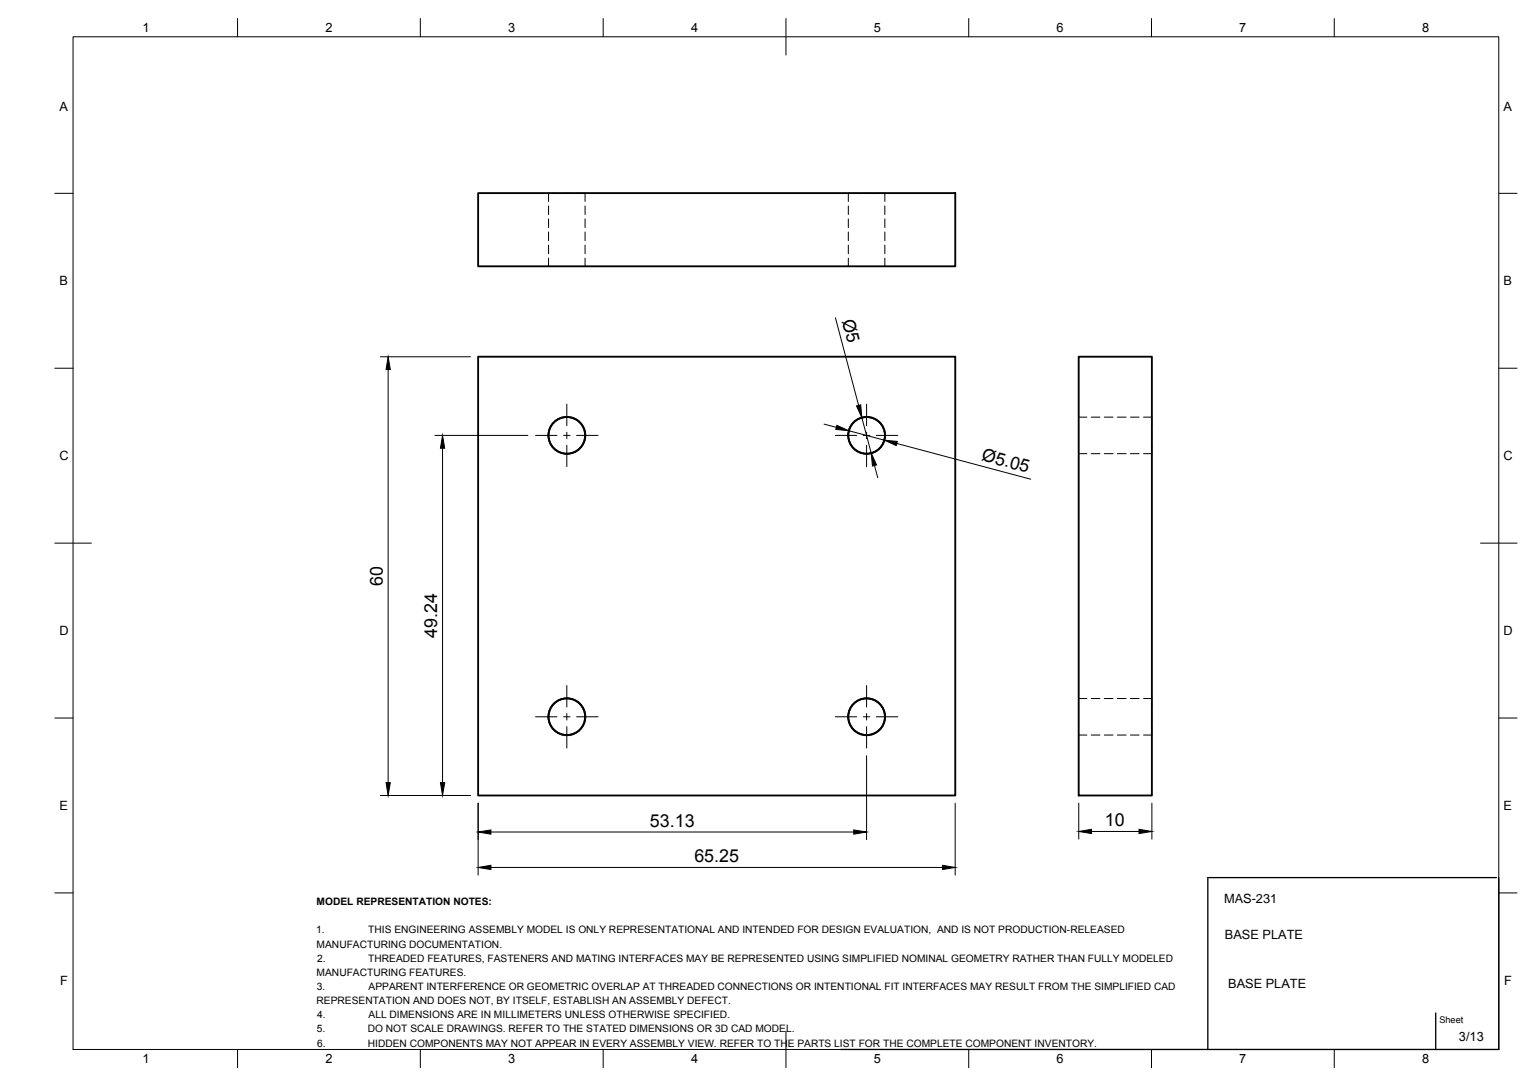
ISO-10303-21;
HEADER;
FILE_DESCRIPTION (('STEP AP214'),
    '1' );
FILE_NAME ( 'Base Plate.step', '2026-10-04T02:08:54', ( '' ), ( '' ), 'STEP AP214', 'Unspecified', '' );
FILE_SCHEMA (( 'AUTOMOTIVE_DESIGN' ));
ENDSEC;
DATA;
#315=EDGE_CURVE ( 'NONE', #5716, #5360, #10980, .T. ) ;
#330=AXIS2_PLACEMENT_3D ( 'NONE', #15898, #1005, #37686 ) ;
#400=CONICAL_SURFACE ( 'NONE', #29553, 0.09842519685039310962, 0.7853981633972314524 ) ;
#581=AXIS2_PLACEMENT_3D ( 'NONE', #37868, #23494, #19160 ) ;
#651=ORIENTED_EDGE ( 'NONE', *, *, #28716, .F. ) ;
#675=DIRECTION ( 'NONE',  ( 0.000000000000000000, 1.000000000000000000, 0.000000000000000000 ) ) ;
#805=AXIS2_PLACEMENT_3D ( 'NONE', #34915, #9017, #31319 ) ;
#889=CARTESIAN_POINT ( 'NONE',  ( 0.8070866141732283561, -0.0009842519685049383633, 0.8559055118110230342 ) ) ;
#932=ORIENTED_EDGE ( 'NONE', *, *, #10243, .T. ) ;
#978=PLANE ( 'NONE',  #26301 ) ;
#991=DIRECTION ( 'NONE',  ( 0.000000000000000000, 1.000000000000000000, 0.000000000000000000 ) ) ;
#1005=DIRECTION ( 'NONE',  ( 0.000000000000000000, 1.000000000000000000, 0.000000000000000000 ) ) ;
#1050=ORIENTED_EDGE ( 'NONE', *, *, #18714, .T. ) ;
#1080=CONICAL_SURFACE ( 'NONE', #330, 0.09842519685039310962, 0.7853981633972314524 ) ;
#1170=VERTEX_POINT ( 'NONE', #7542 ) ;
#1242=VERTEX_POINT ( 'NONE', #23759 ) ;
#1252=EDGE_LOOP ( 'NONE', ( #11130, #15694, #34141, #24810 ) ) ;
#1459=FACE_OUTER_BOUND ( 'NONE', #19089, .T. ) ;
#1546=EDGE_LOOP ( 'NONE', ( #9201, #4846, #43494, #46692 ) ) ;
#1588=ORIENTED_EDGE ( 'NONE', *, *, #46677, .T. ) ;
#1771=DIRECTION ( 'NONE',  ( 0.000000000000000000, 0.000000000000000000, 1.000000000000000000 ) ) ;
#1848=ADVANCED_FACE ( 'NONE', ( #21708 ), #3242, .F. ) ;
#1945=CONICAL_SURFACE ( 'NONE', #26464, 0.09842519685039310962, 0.7853981633972314524 ) ;
#2206=FACE_OUTER_BOUND ( 'NONE', #4838, .T. ) ;
#2223=CARTESIAN_POINT ( 'NONE',  ( 0.8070866141732283561, 0.000000000000000000, 0.7574803149606299524 ) ) ;
#2287=ORIENTED_EDGE ( 'NONE', *, *, #20440, .F. ) ;
#2478=PRODUCT_DEFINITION_CONTEXT ( 'detailed design', #11336, 'design' ) ;
#2480=VERTEX_POINT ( 'NONE', #27806 ) ;
#2571=LINE ( 'NONE', #39233, #13199 ) ;
#2637=ORIENTED_EDGE ( 'NONE', *, *, #8911, .F. ) ;
#2705=ORIENTED_EDGE ( 'NONE', *, *, #4811, .F. ) ;
#2813=DIRECTION ( 'NONE',  ( 0.000000000000000000, 1.000000000000000000, 0.000000000000000000 ) ) ;
#3034=ORIENTED_EDGE ( 'NONE', *, *, #40501, .T. ) ;
#3242=CYLINDRICAL_SURFACE ( 'NONE', #18362, 0.09842519685039310962 ) ;
#3388=( NAMED_UNIT ( * ) SI_UNIT ( $, .STERADIAN. ) SOLID_ANGLE_UNIT ( ) ) ;
#3451=ORIENTED_EDGE ( 'NONE', *, *, #11714, .F. ) ;
#3490=EDGE_LOOP ( 'NONE', ( #8008, #46438, #11694, #3034 ) ) ;
#3519=EDGE_CURVE ( 'NONE', #10456, #24872, #30387, .T. ) ;
#3675=CIRCLE ( 'NONE', #41893, 0.09842519685039310962 ) ;
#3812=FACE_BOUND ( 'NONE', #17412, .T. ) ;
#3834=VERTEX_POINT ( 'NONE', #35885 ) ;
#3929=DIRECTION ( 'NONE',  ( 0.000000000000000000, 1.000000000000000000, 0.000000000000000000 ) ) ;
#3941=LENGTH_MEASURE_WITH_UNIT ( LENGTH_MEASURE( 0.02539999999999999897 ), #37017 ) ;
#3945=DIRECTION ( 'NONE',  ( 0.000000000000000000, 0.000000000000000000, 1.000000000000000000 ) ) ;
#4069=DIRECTION ( 'NONE',  ( 0.000000000000000000, 0.000000000000000000, 1.000000000000000000 ) ) ;
#4078=DIRECTION ( 'NONE',  ( 0.000000000000000000, 0.7071067811867007835, 0.7071067811863941399 ) ) ;
#4150=EDGE_CURVE ( 'NONE', #1170, #31291, #25492, .T. ) ;
#4170=EDGE_LOOP ( 'NONE', ( #24125, #6496, #36526, #10576 ) ) ;
#4195=CIRCLE ( 'NONE', #42468, 0.09940944881889761386 ) ;
#4286=CARTESIAN_POINT ( 'NONE',  ( -1.284448818897637956, -0.3937007874015748254, -1.181102362204724310 ) ) ;
#4382=CARTESIAN_POINT ( 'NONE',  ( 0.8070866141732283561, -0.0009842519685049383633, -0.7574803149606299524 ) ) ;
#4481=AXIS2_PLACEMENT_3D ( 'NONE', #6050, #17084, #13724 ) ;
#4668=EDGE_LOOP ( 'NONE', ( #34347, #651, #38280, #27775 ) ) ;
#4787=CARTESIAN_POINT ( 'NONE',  ( 0.8070866141732283561, -0.0009842519685049383633, -0.8559055118110230342 ) ) ;
#4811=EDGE_CURVE ( 'NONE', #11722, #39584, #46217, .T. ) ;
#4815=DIRECTION ( 'NONE',  ( 1.000000000000000000, -0.000000000000000000, 0.000000000000000000 ) ) ;
#4832=ORIENTED_EDGE ( 'NONE', *, *, #8571, .T. ) ;
#4838=EDGE_LOOP ( 'NONE', ( #34045, #33951, #29727, #22816 ) ) ;
#4846=ORIENTED_EDGE ( 'NONE', *, *, #40501, .F. ) ;
#5141=AXIS2_PLACEMENT_3D ( 'NONE', #9800, #39013, #35676 ) ;
#5145=DIRECTION ( 'NONE',  ( 0.000000000000000000, 1.000000000000000000, 0.000000000000000000 ) ) ;
#5205=ORIENTED_EDGE ( 'NONE', *, *, #25069, .F. ) ;
#5271=CIRCLE ( 'NONE', #26704, 0.09842519685039310962 ) ;
#5360=VERTEX_POINT ( 'NONE', #7812 ) ;
#5579=DIRECTION ( 'NONE',  ( -1.000000000000000000, 0.000000000000000000, 0.000000000000000000 ) ) ;
#5587=AXIS2_PLACEMENT_3D ( 'NONE', #43394, #39329, #25205 ) ;
#5634=DIRECTION ( 'NONE',  ( 0.000000000000000000, 1.000000000000000000, 0.000000000000000000 ) ) ;
#5716=VERTEX_POINT ( 'NONE', #40952 ) ;
#5744=EDGE_CURVE ( 'NONE', #31115, #24872, #37874, .T. ) ;
#5913=EDGE_CURVE ( 'NONE', #14452, #1242, #11460, .T. ) ;
#5977=ADVANCED_FACE ( 'NONE', ( #11706, #44963, #26331, #40892, #22950 ), #18632, .T. ) ;
#6029=DIRECTION ( 'NONE',  ( 0.000000000000000000, 0.000000000000000000, 1.000000000000000000 ) ) ;
#6050=CARTESIAN_POINT ( 'NONE',  ( 0.8070866141732283561, -0.0009842519685049383633, 0.7574803149606299524 ) ) ;
#6143=AXIS2_PLACEMENT_3D ( 'NONE', #30741, #991, #12283 ) ;
#6148=CIRCLE ( 'NONE', #39801, 0.09842519685039310962 ) ;
#6493=ADVANCED_FACE ( 'NONE', ( #34883 ), #1945, .F. ) ;
#6496=ORIENTED_EDGE ( 'NONE', *, *, #25069, .T. ) ;
#6566=VECTOR ( 'NONE', #5579, 39.37007874015748143 ) ;
#6588=DIRECTION ( 'NONE',  ( 0.000000000000000000, 0.000000000000000000, 1.000000000000000000 ) ) ;
#6628=LINE ( 'NONE', #21244, #26508 ) ;
#6675=AXIS2_PLACEMENT_3D ( 'NONE', #36792, #26011, #3945 ) ;
#6892=DIRECTION ( 'NONE',  ( -0.000000000000000000, 1.000000000000000000, -0.000000000000000000 ) ) ;
#7281=DIRECTION ( 'NONE',  ( 0.000000000000000000, 0.000000000000000000, 1.000000000000000000 ) ) ;
#7289=AXIS2_PLACEMENT_3D ( 'NONE', #7614, #32821, #25133 ) ;
#7317=PRODUCT_DEFINITION_SHAPE ( 'NONE', 'NONE',  #36823 ) ;
#7358=FACE_OUTER_BOUND ( 'NONE', #30567, .T. ) ;
#7396=CARTESIAN_POINT ( 'NONE',  ( 0.8070866141732283561, 0.000000000000000000, -0.7574803149606299524 ) ) ;
#7494=ORIENTED_EDGE ( 'NONE', *, *, #46842, .T. ) ;
#7530=CIRCLE ( 'NONE', #20536, 0.09842519685039310962 ) ;
#7542=CARTESIAN_POINT ( 'NONE',  ( -0.8070866141732283561, -0.3937007874015746034, -0.8559055118110230342 ) ) ;
#7568=ADVANCED_FACE ( 'NONE', ( #11132 ), #22840, .T. ) ;
#7614=CARTESIAN_POINT ( 'NONE',  ( -0.8070866141732283561, 0.000000000000000000, 0.7574803149606299524 ) ) ;
#7634=FACE_OUTER_BOUND ( 'NONE', #45486, .T. ) ;
#7663=AXIS2_PLACEMENT_3D ( 'NONE', #26053, #29917, #8526 ) ;
#7737=FACE_OUTER_BOUND ( 'NONE', #25691, .T. ) ;
#7797=EDGE_CURVE ( 'NONE', #28803, #31115, #8610, .T. ) ;
#7798=LINE ( 'NONE', #18816, #17656 ) ;
#7812=CARTESIAN_POINT ( 'NONE',  ( -0.8070866141732283561, 0.000000000000000000, 0.6580708661417323802 ) ) ;
#7880=DIRECTION ( 'NONE',  ( -0.000000000000000000, 1.000000000000000000, 0.000000000000000000 ) ) ;
#7901=EDGE_CURVE ( 'NONE', #15275, #1242, #11102, .T. ) ;
#7933=CARTESIAN_POINT ( 'NONE',  ( 0.8070866141732283561, -0.0009842519685049383633, 0.8559055118110230342 ) ) ;
#8000=CARTESIAN_POINT ( 'NONE',  ( -0.8070866141732283561, 0.000000000000000000, -0.7574803149606299524 ) ) ;
#8008=ORIENTED_EDGE ( 'NONE', *, *, #26812, .F. ) ;
#8058=CARTESIAN_POINT ( 'NONE',  ( 1.284448818897637956, 0.000000000000000000, -1.181102362204724310 ) ) ;
#8059=EDGE_CURVE ( 'NONE', #39837, #14452, #41653, .T. ) ;
#8115=PLANE ( 'NONE',  #11348 ) ;
#8130=UNCERTAINTY_MEASURE_WITH_UNIT (LENGTH_MEASURE( 1.000000000000000082E-05 ), #44890, 'distance_accuracy_value', 'NONE') ;
#8136=DIRECTION ( 'NONE',  ( 0.000000000000000000, 0.000000000000000000, 1.000000000000000000 ) ) ;
#8448=AXIS2_PLACEMENT_3D ( 'NONE', #2223, #41983, #20909 ) ;
#8526=DIRECTION ( 'NONE',  ( 0.000000000000000000, 0.000000000000000000, 1.000000000000000000 ) ) ;
#8571=EDGE_CURVE ( 'NONE', #26504, #25961, #12011, .T. ) ;
#8610=LINE ( 'NONE', #4286, #20278 ) ;
#8677=FACE_OUTER_BOUND ( 'NONE', #35087, .T. ) ;
#8853=ORIENTED_EDGE ( 'NONE', *, *, #11923, .F. ) ;
#8911=EDGE_CURVE ( 'NONE', #25961, #37257, #29546, .T. ) ;
#9017=DIRECTION ( 'NONE',  ( -0.000000000000000000, 1.000000000000000000, -0.000000000000000000 ) ) ;
#9047=ADVANCED_FACE ( 'NONE', ( #25850 ), #40433, .F. ) ;
#9136=DIRECTION ( 'NONE',  ( -0.000000000000000000, 1.000000000000000000, -0.000000000000000000 ) ) ;
#9137=AXIS2_PLACEMENT_3D ( 'NONE', #36669, #14627, #21570 ) ;
#9201=ORIENTED_EDGE ( 'NONE', *, *, #27851, .F. ) ;
#9223=AXIS2_PLACEMENT_3D ( 'NONE', #8000, #18549, #29403 ) ;
#9407=ORIENTED_EDGE ( 'NONE', *, *, #4150, .F. ) ;
#9658=SHAPE_DEFINITION_REPRESENTATION ( #7317, #30762 ) ;
#9710=EDGE_CURVE ( 'NONE', #18061, #11722, #40144, .T. ) ;
#9759=DIRECTION ( 'NONE',  ( 0.000000000000000000, 0.000000000000000000, -1.000000000000000000 ) ) ;
#9800=CARTESIAN_POINT ( 'NONE',  ( 0.8070866141732283561, -0.0009842519685049383633, 0.7574803149606299524 ) ) ;
#9852=ORIENTED_EDGE ( 'NONE', *, *, #7901, .F. ) ;
#10204=CARTESIAN_POINT ( 'NONE',  ( 0.8070866141732283561, -0.3937007874015746034, -0.7574803149606299524 ) ) ;
#10243=EDGE_CURVE ( 'NONE', #44955, #14452, #31944, .T. ) ;
#10358=EDGE_LOOP ( 'NONE', ( #22529, #42334, #12122, #27521 ) ) ;
#10359=EDGE_CURVE ( 'NONE', #22756, #27408, #46200, .T. ) ;
#10456=VERTEX_POINT ( 'NONE', #22399 ) ;
#10576=ORIENTED_EDGE ( 'NONE', *, *, #46842, .F. ) ;
#10585=CARTESIAN_POINT ( 'NONE',  ( -0.8070866141732283561, -0.3937007874015746034, 0.7574803149606299524 ) ) ;
#10681=EDGE_CURVE ( 'NONE', #20094, #24250, #43403, .T. ) ;
#10719=DIRECTION ( 'NONE',  ( 8.659560562353054383E-17, 0.7071067811867007835, -0.7071067811863941399 ) ) ;
#10725=EDGE_CURVE ( 'NONE', #22756, #28803, #40345, .T. ) ;
#10805=MECHANICAL_DESIGN_GEOMETRIC_PRESENTATION_REPRESENTATION('',(#19186),#41362);
#10835=DIRECTION ( 'NONE',  ( 1.000000000000000000, 0.000000000000000000, 0.000000000000000000 ) ) ;
#10869=DIRECTION ( 'NONE',  ( 0.000000000000000000, 0.000000000000000000, 1.000000000000000000 ) ) ;
#10980=CIRCLE ( 'NONE', #37859, 0.09940944881889761386 ) ;
#11020=DIRECTION ( 'NONE',  ( 8.659560562353054383E-17, 0.7071067811867007835, -0.7071067811863941399 ) ) ;
#11049=ORIENTED_EDGE ( 'NONE', *, *, #43540, .F. ) ;
#11074=EDGE_CURVE ( 'NONE', #29015, #39837, #11313, .T. ) ;
#11102=CIRCLE ( 'NONE', #43217, 0.09940944881889761386 ) ;
#11130=ORIENTED_EDGE ( 'NONE', *, *, #20351, .F. ) ;
#11132=FACE_OUTER_BOUND ( 'NONE', #12538, .T. ) ;
#11176=ORIENTED_EDGE ( 'NONE', *, *, #19700, .F. ) ;
#11220=CARTESIAN_POINT ( 'NONE',  ( 0.8070866141732283561, 0.000000000000000000, 0.8559055118110230342 ) ) ;
#11313=CIRCLE ( 'NONE', #6675, 0.09842519685039310962 ) ;
#11336=APPLICATION_CONTEXT ( 'automotive_design' ) ;
#11348=AXIS2_PLACEMENT_3D ( 'NONE', #33797, #7880, #15576 ) ;
#11385=CARTESIAN_POINT ( 'NONE',  ( 1.284448818897637956, -0.3937007874015748254, -1.181102362204724310 ) ) ;
#11450=AXIS2_PLACEMENT_3D ( 'NONE', #22352, #13997, #7281 ) ;
#11460=LINE ( 'NONE', #25845, #21062 ) ;
#11694=ORIENTED_EDGE ( 'NONE', *, *, #16527, .T. ) ;
#11706=FACE_BOUND ( 'NONE', #31447, .T. ) ;
#11714=EDGE_CURVE ( 'NONE', #32806, #13348, #3675, .T. ) ;
#11722=VERTEX_POINT ( 'NONE', #43133 ) ;
#11838=LINE ( 'NONE', #34587, #6566 ) ;
#11889=VECTOR ( 'NONE', #14058, 39.37007874015748143 ) ;
#11923=EDGE_CURVE ( 'NONE', #26504, #47218, #15149, .T. ) ;
#11943=FACE_OUTER_BOUND ( 'NONE', #3490, .T. ) ;
#12011=LINE ( 'NONE', #4787, #14204 ) ;
#12089=ORIENTED_EDGE ( 'NONE', *, *, #8059, .F. ) ;
#12122=ORIENTED_EDGE ( 'NONE', *, *, #17641, .T. ) ;
#12174=DIRECTION ( 'NONE',  ( -0.000000000000000000, 1.000000000000000000, 0.000000000000000000 ) ) ;
#12192=CARTESIAN_POINT ( 'NONE',  ( -0.8070866141732283561, -0.0009842519685049383633, 0.8559055118110230342 ) ) ;
#12197=CYLINDRICAL_SURFACE ( 'NONE', #24627, 0.09842519685039310962 ) ;
#12201=EDGE_CURVE ( 'NONE', #36286, #31518, #7530, .T. ) ;
#12283=DIRECTION ( 'NONE',  ( 0.000000000000000000, 0.000000000000000000, 1.000000000000000000 ) ) ;
#12373=ORIENTED_EDGE ( 'NONE', *, *, #22828, .F. ) ;
#12375=EDGE_CURVE ( 'NONE', #47218, #37257, #18468, .T. ) ;
#12379=AXIS2_PLACEMENT_3D ( 'NONE', #32536, #33483, #25809 ) ;
#12420=AXIS2_PLACEMENT_3D ( 'NONE', #32416, #39325, #14656 ) ;
#12507=DIRECTION ( 'NONE',  ( 0.000000000000000000, 0.7071067811867007835, 0.7071067811863941399 ) ) ;
#12538=EDGE_LOOP ( 'NONE', ( #42275, #17973, #13010, #43115 ) ) ;
#12632=DIRECTION ( 'NONE',  ( 0.000000000000000000, 0.000000000000000000, -1.000000000000000000 ) ) ;
#12979=CARTESIAN_POINT ( 'NONE',  ( 1.284448818897637956, -0.3937007874015748254, 1.181102362204724310 ) ) ;
#13010=ORIENTED_EDGE ( 'NONE', *, *, #10725, .T. ) ;
#13076=ORIENTED_EDGE ( 'NONE', *, *, #8911, .T. ) ;
#13199=VECTOR ( 'NONE', #38781, 39.37007874015748143 ) ;
#13203=CIRCLE ( 'NONE', #45310, 0.09940944881889761386 ) ;
#13257=CYLINDRICAL_SURFACE ( 'NONE', #24915, 0.09842519685039310962 ) ;
#13309=EDGE_LOOP ( 'NONE', ( #34696, #24463, #14277, #2705 ) ) ;
#13348=VERTEX_POINT ( 'NONE', #24149 ) ;
#13360=ORIENTED_EDGE ( 'NONE', *, *, #44670, .T. ) ;
#13364=EDGE_LOOP ( 'NONE', ( #12089, #19872, #15320, #932 ) ) ;
#13405=EDGE_CURVE ( 'NONE', #3834, #22756, #46869, .T. ) ;
#13497=ORIENTED_EDGE ( 'NONE', *, *, #19700, .T. ) ;
#13698=ORIENTED_EDGE ( 'NONE', *, *, #39533, .F. ) ;
#13709=CARTESIAN_POINT ( 'NONE',  ( -0.8070866141732283561, 0.000000000000000000, -0.7574803149606299524 ) ) ;
#13724=DIRECTION ( 'NONE',  ( 0.000000000000000000, 0.000000000000000000, 1.000000000000000000 ) ) ;
#13782=VECTOR ( 'NONE', #6892, 39.37007874015748143 ) ;
#13997=DIRECTION ( 'NONE',  ( -0.000000000000000000, 1.000000000000000000, -0.000000000000000000 ) ) ;
#14005=CARTESIAN_POINT ( 'NONE',  ( -0.8070866141732283561, -0.3937007874015746034, -0.7574803149606299524 ) ) ;
#14054=CARTESIAN_POINT ( 'NONE',  ( 1.284448818897637956, -0.3937007874015748254, 1.181102362204724310 ) ) ;
#14058=DIRECTION ( 'NONE',  ( -0.000000000000000000, 1.000000000000000000, -0.000000000000000000 ) ) ;
#14204=VECTOR ( 'NONE', #40958, 39.37007874015748854 ) ;
#14277=ORIENTED_EDGE ( 'NONE', *, *, #20440, .T. ) ;
#14409=ADVANCED_FACE ( 'NONE', ( #7737 ), #17827, .F. ) ;
#14452=VERTEX_POINT ( 'NONE', #22120 ) ;
#14627=DIRECTION ( 'NONE',  ( 0.000000000000000000, 1.000000000000000000, 0.000000000000000000 ) ) ;
#14629=ORIENTED_EDGE ( 'NONE', *, *, #22828, .T. ) ;
#14653=AXIS2_PLACEMENT_3D ( 'NONE', #16888, #5634, #45630 ) ;
#14656=DIRECTION ( 'NONE',  ( 0.000000000000000000, 0.000000000000000000, 1.000000000000000000 ) ) ;
#14766=( GEOMETRIC_REPRESENTATION_CONTEXT ( 3 ) GLOBAL_UNCERTAINTY_ASSIGNED_CONTEXT ( ( #32575 ) ) GLOBAL_UNIT_ASSIGNED_CONTEXT ( ( #46283, #42665, #3388 ) ) REPRESENTATION_CONTEXT ( 'NONE', 'WORKASPACE' ) ) ;
#14804=CLOSED_SHELL ( 'NONE', ( #31070, #18070, #45753, #6493, #9047, #14409, #42647, #19306, #16260, #45323, #7568, #24097, #26805, #5977, #31234, #16585, #35710, #1848, #42716, #25765, #41567, #28656 ) ) ;
#14846=CARTESIAN_POINT ( 'NONE',  ( -1.284448818897637956, -0.3937007874015748254, 1.181102362204724310 ) ) ;
#14989=DIRECTION ( 'NONE',  ( -1.000000000000000000, 0.000000000000000000, 0.000000000000000000 ) ) ;
#15029=PLANE ( 'NONE',  #12379 ) ;
#15036=DIRECTION ( 'NONE',  ( 0.000000000000000000, 1.000000000000000000, 0.000000000000000000 ) ) ;
#15056=ORIENTED_EDGE ( 'NONE', *, *, #5913, .T. ) ;
#15149=CIRCLE ( 'NONE', #581, 0.09842519685039310962 ) ;
#15212=DIRECTION ( 'NONE',  ( 0.000000000000000000, 1.000000000000000000, 0.000000000000000000 ) ) ;
#15252=ORIENTED_EDGE ( 'NONE', *, *, #17641, .F. ) ;
#15275=VERTEX_POINT ( 'NONE', #28091 ) ;
#15315=CARTESIAN_POINT ( 'NONE',  ( -0.8070866141732283561, -0.3937007874015746034, -0.6590551181102368705 ) ) ;
#15320=ORIENTED_EDGE ( 'NONE', *, *, #30247, .T. ) ;
#15348=CIRCLE ( 'NONE', #8448, 0.09940944881889761386 ) ;
#15352=AXIS2_PLACEMENT_3D ( 'NONE', #18404, #26565, #22948 ) ;
#15387=DIRECTION ( 'NONE',  ( 0.000000000000000000, 0.000000000000000000, 1.000000000000000000 ) ) ;
#15576=DIRECTION ( 'NONE',  ( 0.000000000000000000, -0.000000000000000000, 1.000000000000000000 ) ) ;
#15694=ORIENTED_EDGE ( 'NONE', *, *, #30183, .T. ) ;
#15854=ORIENTED_EDGE ( 'NONE', *, *, #41961, .T. ) ;
#15897=ORIENTED_EDGE ( 'NONE', *, *, #16527, .F. ) ;
#15898=CARTESIAN_POINT ( 'NONE',  ( -0.8070866141732283561, -0.0009842519685049383633, 0.7574803149606299524 ) ) ;
#15935=VECTOR ( 'NONE', #3929, 39.37007874015748143 ) ;
#16087=ORIENTED_EDGE ( 'NONE', *, *, #19646, .T. ) ;
#16138=CARTESIAN_POINT ( 'NONE',  ( 0.8070866141732283561, -0.0009842519685049383633, -0.6590551181102368705 ) ) ;
#16176=CIRCLE ( 'NONE', #805, 0.09842519685039310962 ) ;
#16184=CONICAL_SURFACE ( 'NONE', #26125, 0.09842519685039310962, 0.7853981633972314524 ) ;
#16260=ADVANCED_FACE ( 'NONE', ( #11943 ), #37084, .T. ) ;
#16305=CARTESIAN_POINT ( 'NONE',  ( -0.8070866141732283561, -0.0009842519685049383633, 0.7574803149606299524 ) ) ;
#16485=DIRECTION ( 'NONE',  ( 0.000000000000000000, 0.000000000000000000, 1.000000000000000000 ) ) ;
#16527=EDGE_CURVE ( 'NONE', #31115, #3834, #7798, .T. ) ;
#16529=ORIENTED_EDGE ( 'NONE', *, *, #16885, .F. ) ;
#16585=ADVANCED_FACE ( 'NONE', ( #38454 ), #16657, .F. ) ;
#16623=EDGE_LOOP ( 'NONE', ( #11176, #44889, #39910, #2287 ) ) ;
#16657=CYLINDRICAL_SURFACE ( 'NONE', #43646, 0.09842519685039310962 ) ;
#16846=FACE_OUTER_BOUND ( 'NONE', #10358, .T. ) ;
#16870=AXIS2_PLACEMENT_3D ( 'NONE', #13709, #33314, #37108 ) ;
#16885=EDGE_CURVE ( 'NONE', #39837, #29015, #6148, .T. ) ;
#16888=CARTESIAN_POINT ( 'NONE',  ( 0.8070866141732283561, -0.0009842519685049383633, -0.7574803149606299524 ) ) ;
#17019=CARTESIAN_POINT ( 'NONE',  ( -1.284448818897637956, 0.000000000000000000, 1.181102362204724310 ) ) ;
#17084=DIRECTION ( 'NONE',  ( 0.000000000000000000, 1.000000000000000000, 0.000000000000000000 ) ) ;
#17092=ORIENTED_EDGE ( 'NONE', *, *, #20351, .T. ) ;
#17162=DIRECTION ( 'NONE',  ( 0.000000000000000000, 0.000000000000000000, 1.000000000000000000 ) ) ;
#17412=EDGE_LOOP ( 'NONE', ( #25328, #41077 ) ) ;
#17415=DIRECTION ( 'NONE',  ( -0.000000000000000000, 1.000000000000000000, -0.000000000000000000 ) ) ;
#17551=EDGE_LOOP ( 'NONE', ( #35799, #16087 ) ) ;
#17621=AXIS2_PLACEMENT_3D ( 'NONE', #28129, #675, #22744 ) ;
#17628=ORIENTED_EDGE ( 'NONE', *, *, #46027, .T. ) ;
#17641=EDGE_CURVE ( 'NONE', #44955, #15275, #40738, .T. ) ;
#17648=CARTESIAN_POINT ( 'NONE',  ( -0.8070866141732283561, 0.000000000000000000, 0.8559055118110230342 ) ) ;
#17656=VECTOR ( 'NONE', #33472, 39.37007874015748143 ) ;
#17827=CYLINDRICAL_SURFACE ( 'NONE', #11450, 0.09842519685039310962 ) ;
#17870=CARTESIAN_POINT ( 'NONE',  ( -0.8070866141732283561, 0.000000000000000000, 0.7574803149606299524 ) ) ;
#17891=FACE_OUTER_BOUND ( 'NONE', #4668, .T. ) ;
#17973=ORIENTED_EDGE ( 'NONE', *, *, #10359, .F. ) ;
#18061=VERTEX_POINT ( 'NONE', #25870 ) ;
#18070=ADVANCED_FACE ( 'NONE', ( #44990 ), #16184, .F. ) ;
#18083=DIRECTION ( 'NONE',  ( 0.000000000000000000, 0.000000000000000000, 1.000000000000000000 ) ) ;
#18274=CARTESIAN_POINT ( 'NONE',  ( 1.284448818897637956, -0.3937007874015748254, -1.181102362204724310 ) ) ;
#18362=AXIS2_PLACEMENT_3D ( 'NONE', #17870, #25309, #17162 ) ;
#18404=CARTESIAN_POINT ( 'NONE',  ( -1.284448818897637956, -0.3937007874015748254, 1.181102362204724310 ) ) ;
#18468=LINE ( 'NONE', #44100, #47325 ) ;
#18477=CIRCLE ( 'NONE', #7663, 0.09842519685039310962 ) ;
#18536=DIRECTION ( 'NONE',  ( 0.000000000000000000, 0.000000000000000000, -1.000000000000000000 ) ) ;
#18549=DIRECTION ( 'NONE',  ( -0.000000000000000000, 1.000000000000000000, -0.000000000000000000 ) ) ;
#18632=PLANE ( 'NONE',  #43266 ) ;
#18639=AXIS2_PLACEMENT_3D ( 'NONE', #40445, #37335, #26349 ) ;
#18660=DIRECTION ( 'NONE',  ( 0.000000000000000000, 1.000000000000000000, 0.000000000000000000 ) ) ;
#18714=EDGE_CURVE ( 'NONE', #14452, #44955, #18477, .T. ) ;
#18719=CARTESIAN_POINT ( 'NONE',  ( 0.8070866141732283561, -0.3937007874015746034, -0.7574803149606299524 ) ) ;
#18783=CYLINDRICAL_SURFACE ( 'NONE', #9223, 0.09842519685039310962 ) ;
#18798=PRODUCT ( 'Base Plate', 'Base Plate', '', ( #24502 ) ) ;
#18816=CARTESIAN_POINT ( 'NONE',  ( -1.284448818897637956, -0.3937007874015748254, 1.181102362204724310 ) ) ;
#18853=LINE ( 'NONE', #11220, #23743 ) ;
#19080=CARTESIAN_POINT ( 'NONE',  ( 0.8070866141732283561, -0.3937007874015746034, -0.8559055118110230342 ) ) ;
#19089=EDGE_LOOP ( 'NONE', ( #34703, #15056, #9852, #15252 ) ) ;
#19126=DIRECTION ( 'NONE',  ( 0.000000000000000000, 0.000000000000000000, 1.000000000000000000 ) ) ;
#19160=DIRECTION ( 'NONE',  ( 0.000000000000000000, 0.000000000000000000, 1.000000000000000000 ) ) ;
#19186=STYLED_ITEM ( 'NONE', ( #25777 ), #20717 ) ;
#19306=ADVANCED_FACE ( 'NONE', ( #22859 ), #18783, .F. ) ;
#19399=CIRCLE ( 'NONE', #18639, 0.09842519685039310962 ) ;
#19491=AXIS2_PLACEMENT_3D ( 'NONE', #29389, #18536, #37453 ) ;
#19646=EDGE_CURVE ( 'NONE', #1242, #15275, #15348, .T. ) ;
#19649=CARTESIAN_POINT ( 'NONE',  ( -1.284448818897637956, -0.3937007874015748254, 1.181102362204724310 ) ) ;
#19700=EDGE_CURVE ( 'NONE', #18061, #2480, #38282, .T. ) ;
#19768=DIRECTION ( 'NONE',  ( 0.000000000000000000, 0.000000000000000000, 1.000000000000000000 ) ) ;
#19872=ORIENTED_EDGE ( 'NONE', *, *, #11074, .F. ) ;
#20094=VERTEX_POINT ( 'NONE', #19080 ) ;
#20200=CARTESIAN_POINT ( 'NONE',  ( -1.284448818897637956, -0.3937007874015748254, -1.181102362204724310 ) ) ;
#20278=VECTOR ( 'NONE', #4069, 39.37007874015748143 ) ;
#20297=DIRECTION ( 'NONE',  ( 0.000000000000000000, -1.000000000000000000, -0.000000000000000000 ) ) ;
#20351=EDGE_CURVE ( 'NONE', #13348, #32806, #16176, .T. ) ;
#20440=EDGE_CURVE ( 'NONE', #2480, #39584, #29168, .T. ) ;
#20536=AXIS2_PLACEMENT_3D ( 'NONE', #16305, #31865, #42134 ) ;
#20619=CIRCLE ( 'NONE', #9137, 0.09842519685039310962 ) ;
#20717=MANIFOLD_SOLID_BREP ( 'Base Plate', #14804 ) ;
#20860=AXIS2_PLACEMENT_3D ( 'NONE', #25692, #32652, #10835 ) ;
#20909=DIRECTION ( 'NONE',  ( 0.000000000000000000, 0.000000000000000000, 1.000000000000000000 ) ) ;
#21062=VECTOR ( 'NONE', #33998, 39.37007874015748854 ) ;
#21118=CIRCLE ( 'NONE', #27293, 0.09842519685039310962 ) ;
#21215=VECTOR ( 'NONE', #14989, 39.37007874015748143 ) ;
#21234=ORIENTED_EDGE ( 'NONE', *, *, #12375, .F. ) ;
#21244=CARTESIAN_POINT ( 'NONE',  ( -0.8070866141732283561, 0.000000000000000000, -0.6590551181102368705 ) ) ;
#21367=CYLINDRICAL_SURFACE ( 'NONE', #16870, 0.09842519685039310962 ) ;
#21570=DIRECTION ( 'NONE',  ( 0.000000000000000000, 0.000000000000000000, 1.000000000000000000 ) ) ;
#21672=DIRECTION ( 'NONE',  ( -0.000000000000000000, 1.000000000000000000, -0.000000000000000000 ) ) ;
#21708=FACE_OUTER_BOUND ( 'NONE', #43993, .T. ) ;
#21834=ORIENTED_EDGE ( 'NONE', *, *, #12201, .F. ) ;
#21907=DIRECTION ( 'NONE',  ( 0.000000000000000000, 0.000000000000000000, 1.000000000000000000 ) ) ;
#22008=AXIS2_PLACEMENT_3D ( 'NONE', #10204, #39406, #6588 ) ;
#22120=CARTESIAN_POINT ( 'NONE',  ( 0.8070866141732283561, -0.0009842519685049383633, 0.6590551181102368705 ) ) ;
#22280=DIRECTION ( 'NONE',  ( 0.000000000000000000, 0.000000000000000000, 1.000000000000000000 ) ) ;
#22352=CARTESIAN_POINT ( 'NONE',  ( 0.8070866141732283561, 0.000000000000000000, 0.7574803149606299524 ) ) ;
#22390=SURFACE_STYLE_USAGE ( .BOTH. , #30341 ) ;
#22399=CARTESIAN_POINT ( 'NONE',  ( -1.284448818897637956, 0.000000000000000000, -1.181102362204724310 ) ) ;
#22420=ORIENTED_EDGE ( 'NONE', *, *, #12375, .T. ) ;
#22529=ORIENTED_EDGE ( 'NONE', *, *, #5913, .F. ) ;
#22724=VECTOR ( 'NONE', #10719, 39.37007874015748854 ) ;
#22725=EDGE_CURVE ( 'NONE', #5360, #5716, #13203, .T. ) ;
#22744=DIRECTION ( 'NONE',  ( 0.000000000000000000, 0.000000000000000000, 1.000000000000000000 ) ) ;
#22756=VERTEX_POINT ( 'NONE', #18274 ) ;
#22816=ORIENTED_EDGE ( 'NONE', *, *, #34489, .F. ) ;
#22828=EDGE_CURVE ( 'NONE', #1170, #18061, #33160, .T. ) ;
#22840=PLANE ( 'NONE',  #19491 ) ;
#22859=FACE_OUTER_BOUND ( 'NONE', #34603, .T. ) ;
#22948=DIRECTION ( 'NONE',  ( 1.000000000000000000, 0.000000000000000000, -0.000000000000000000 ) ) ;
#22950=FACE_OUTER_BOUND ( 'NONE', #38338, .T. ) ;
#22967=LINE ( 'NONE', #12192, #44518 ) ;
#22978=DIRECTION ( 'NONE',  ( 1.000000000000000000, 0.000000000000000000, 0.000000000000000000 ) ) ;
#23117=DIRECTION ( 'NONE',  ( -0.000000000000000000, 1.000000000000000000, -0.000000000000000000 ) ) ;
#23337=CARTESIAN_POINT ( 'NONE',  ( -0.8070866141732283561, -0.0009842519685049383633, 0.8559055118110230342 ) ) ;
#23494=DIRECTION ( 'NONE',  ( 0.000000000000000000, 1.000000000000000000, 0.000000000000000000 ) ) ;
#23606=DIRECTION ( 'NONE',  ( 0.000000000000000000, 0.000000000000000000, 1.000000000000000000 ) ) ;
#23633=LINE ( 'NONE', #26771, #29018 ) ;
#23743=VECTOR ( 'NONE', #33757, 39.37007874015748143 ) ;
#23759=CARTESIAN_POINT ( 'NONE',  ( 0.8070866141732283561, 0.000000000000000000, 0.6580708661417323802 ) ) ;
#23862=CARTESIAN_POINT ( 'NONE',  ( 0.8070866141732283561, 0.000000000000000000, -0.8568897637795275246 ) ) ;
#23928=VECTOR ( 'NONE', #9136, 39.37007874015748143 ) ;
#24097=ADVANCED_FACE ( 'NONE', ( #30963 ), #978, .T. ) ;
#24125=ORIENTED_EDGE ( 'NONE', *, *, #29501, .F. ) ;
#24149=CARTESIAN_POINT ( 'NONE',  ( -0.8070866141732283561, -0.3937007874015746034, 0.6590551181102368705 ) ) ;
#24250=VERTEX_POINT ( 'NONE', #47409 ) ;
#24270=FACE_OUTER_BOUND ( 'NONE', #13309, .T. ) ;
#24463=ORIENTED_EDGE ( 'NONE', *, *, #25166, .F. ) ;
#24502=PRODUCT_CONTEXT ( 'NONE', #29442, 'mechanical' ) ;
#24627=AXIS2_PLACEMENT_3D ( 'NONE', #42099, #37580, #19126 ) ;
#24810=ORIENTED_EDGE ( 'NONE', *, *, #44670, .F. ) ;
#24872=VERTEX_POINT ( 'NONE', #17019 ) ;
#24885=CARTESIAN_POINT ( 'NONE',  ( -0.8070866141732283561, 0.000000000000000000, 0.6590551181102368705 ) ) ;
#24915=AXIS2_PLACEMENT_3D ( 'NONE', #45341, #31231, #6029 ) ;
#25069=EDGE_CURVE ( 'NONE', #31518, #5360, #44513, .T. ) ;
#25133=DIRECTION ( 'NONE',  ( 0.000000000000000000, 0.000000000000000000, 1.000000000000000000 ) ) ;
#25166=EDGE_CURVE ( 'NONE', #2480, #18061, #19399, .T. ) ;
#25205=DIRECTION ( 'NONE',  ( 0.000000000000000000, 0.000000000000000000, 1.000000000000000000 ) ) ;
#25309=DIRECTION ( 'NONE',  ( -0.000000000000000000, 1.000000000000000000, -0.000000000000000000 ) ) ;
#25328=ORIENTED_EDGE ( 'NONE', *, *, #11074, .T. ) ;
#25492=CIRCLE ( 'NONE', #5587, 0.09842519685039310962 ) ;
#25691=EDGE_LOOP ( 'NONE', ( #16529, #27816, #1050, #45866 ) ) ;
#25692=CARTESIAN_POINT ( 'NONE',  ( 0.000000000000000000, 0.000000000000000000, 0.000000000000000000 ) ) ;
#25765=ADVANCED_FACE ( 'NONE', ( #7358 ), #34784, .F. ) ;
#25777=PRESENTATION_STYLE_ASSIGNMENT (( #22390 ) ) ;
#25809=DIRECTION ( 'NONE',  ( 0.000000000000000000, 0.000000000000000000, 1.000000000000000000 ) ) ;
#25845=CARTESIAN_POINT ( 'NONE',  ( 0.8070866141732283561, -0.0009842519685049383633, 0.6590551181102368705 ) ) ;
#25850=FACE_OUTER_BOUND ( 'NONE', #1252, .T. ) ;
#25870=CARTESIAN_POINT ( 'NONE',  ( -0.8070866141732283561, -0.0009842519685049383633, -0.8559055118110230342 ) ) ;
#25961=VERTEX_POINT ( 'NONE', #23862 ) ;
#26011=DIRECTION ( 'NONE',  ( -0.000000000000000000, 1.000000000000000000, -0.000000000000000000 ) ) ;
#26053=CARTESIAN_POINT ( 'NONE',  ( 0.8070866141732283561, -0.0009842519685049383633, 0.7574803149606299524 ) ) ;
#26125=AXIS2_PLACEMENT_3D ( 'NONE', #41383, #18660, #33550 ) ;
#26301=AXIS2_PLACEMENT_3D ( 'NONE', #12979, #4815, #41694 ) ;
#26331=FACE_BOUND ( 'NONE', #33025, .T. ) ;
#26349=DIRECTION ( 'NONE',  ( 0.000000000000000000, 0.000000000000000000, 1.000000000000000000 ) ) ;
#26360=FACE_OUTER_BOUND ( 'NONE', #38562, .T. ) ;
#26425=CARTESIAN_POINT ( 'NONE',  ( -0.8070866141732283561, 0.000000000000000000, 0.7574803149606299524 ) ) ;
#26464=AXIS2_PLACEMENT_3D ( 'NONE', #37987, #5145, #19768 ) ;
#26504=VERTEX_POINT ( 'NONE', #34361 ) ;
#26508=VECTOR ( 'NONE', #17415, 39.37007874015748143 ) ;
#26565=DIRECTION ( 'NONE',  ( 0.000000000000000000, 0.000000000000000000, 1.000000000000000000 ) ) ;
#26679=ORIENTED_EDGE ( 'NONE', *, *, #12201, .T. ) ;
#26704=AXIS2_PLACEMENT_3D ( 'NONE', #4382, #15212, #18083 ) ;
#26771=CARTESIAN_POINT ( 'NONE',  ( 0.8070866141732283561, 0.000000000000000000, -0.8559055118110230342 ) ) ;
#26798=DIRECTION ( 'NONE',  ( 0.000000000000000000, -0.000000000000000000, 1.000000000000000000 ) ) ;
#26803=CARTESIAN_POINT ( 'NONE',  ( -0.8070866141732283561, 0.000000000000000000, -0.7574803149606299524 ) ) ;
#26805=ADVANCED_FACE ( 'NONE', ( #30215, #3812, #33082, #44760, #26360 ), #8115, .F. ) ;
#26812=EDGE_CURVE ( 'NONE', #24872, #32629, #44065, .T. ) ;
#26976=ORIENTED_EDGE ( 'NONE', *, *, #25166, .T. ) ;
#27023=ORIENTED_EDGE ( 'NONE', *, *, #26812, .T. ) ;
#27165=AXIS2_PLACEMENT_3D ( 'NONE', #33260, #15036, #40391 ) ;
#27293=AXIS2_PLACEMENT_3D ( 'NONE', #18719, #36486, #15387 ) ;
#27401=ADVANCED_BREP_SHAPE_REPRESENTATION ( 'Base Plate', ( #20717, #20860 ), #14766 ) ;
#27408=VERTEX_POINT ( 'NONE', #8058 ) ;
#27448=VECTOR ( 'NONE', #22978, 39.37007874015748143 ) ;
#27521=ORIENTED_EDGE ( 'NONE', *, *, #19646, .F. ) ;
#27547=FACE_OUTER_BOUND ( 'NONE', #13364, .T. ) ;
#27705=EDGE_CURVE ( 'NONE', #20094, #26504, #23633, .T. ) ;
#27775=ORIENTED_EDGE ( 'NONE', *, *, #5744, .T. ) ;
#27806=CARTESIAN_POINT ( 'NONE',  ( -0.8070866141732283561, -0.0009842519685049383633, -0.6590551181102368705 ) ) ;
#27816=ORIENTED_EDGE ( 'NONE', *, *, #8059, .T. ) ;
#27851=EDGE_CURVE ( 'NONE', #32629, #27408, #45175, .T. ) ;
#28062=CARTESIAN_POINT ( 'NONE',  ( -0.8070866141732283561, 0.000000000000000000, -0.7574803149606299524 ) ) ;
#28091=CARTESIAN_POINT ( 'NONE',  ( 0.8070866141732283561, 0.000000000000000000, 0.8568897637795275246 ) ) ;
#28129=CARTESIAN_POINT ( 'NONE',  ( -0.8070866141732283561, -0.0009842519685049383633, -0.7574803149606299524 ) ) ;
#28155=EDGE_CURVE ( 'NONE', #47218, #26504, #5271, .T. ) ;
#28243=VECTOR ( 'NONE', #12632, 39.37007874015748143 ) ;
#28493=CIRCLE ( 'NONE', #45279, 0.09842519685039310962 ) ;
#28613=ORIENTED_EDGE ( 'NONE', *, *, #11714, .T. ) ;
#28656=ADVANCED_FACE ( 'NONE', ( #16846 ), #32103, .F. ) ;
#28716=EDGE_CURVE ( 'NONE', #28803, #10456, #39585, .T. ) ;
#28803=VERTEX_POINT ( 'NONE', #29098 ) ;
#29015=VERTEX_POINT ( 'NONE', #40749 ) ;
#29018=VECTOR ( 'NONE', #38243, 39.37007874015748143 ) ;
#29098=CARTESIAN_POINT ( 'NONE',  ( -1.284448818897637956, -0.3937007874015748254, -1.181102362204724310 ) ) ;
#29168=LINE ( 'NONE', #39409, #45206 ) ;
#29389=CARTESIAN_POINT ( 'NONE',  ( 1.284448818897637956, -0.3937007874015748254, -1.181102362204724310 ) ) ;
#29403=DIRECTION ( 'NONE',  ( 0.000000000000000000, 0.000000000000000000, 1.000000000000000000 ) ) ;
#29417=( NAMED_UNIT ( * ) PLANE_ANGLE_UNIT ( ) SI_UNIT ( $, .RADIAN. ) ) ;
#29442=APPLICATION_CONTEXT ( 'automotive_design' ) ;
#29443=EDGE_LOOP ( 'NONE', ( #1588, #13076 ) ) ;
#29501=EDGE_CURVE ( 'NONE', #31518, #36286, #20619, .T. ) ;
#29538=DIRECTION ( 'NONE',  ( -0.000000000000000000, 1.000000000000000000, -0.000000000000000000 ) ) ;
#29546=CIRCLE ( 'NONE', #40951, 0.09940944881889761386 ) ;
#29553=AXIS2_PLACEMENT_3D ( 'NONE', #38640, #46049, #38401 ) ;
#29647=DIRECTION ( 'NONE',  ( 0.000000000000000000, 0.000000000000000000, 1.000000000000000000 ) ) ;
#29727=ORIENTED_EDGE ( 'NONE', *, *, #11923, .T. ) ;
#29917=DIRECTION ( 'NONE',  ( 0.000000000000000000, 1.000000000000000000, 0.000000000000000000 ) ) ;
#30000=CARTESIAN_POINT ( 'NONE',  ( 0.8070866141732283561, 0.000000000000000000, 0.7574803149606299524 ) ) ;
#30103=LINE ( 'NONE', #41041, #15935 ) ;
#30115=CARTESIAN_POINT ( 'NONE',  ( 0.8070866141732283561, -0.3937007874015746034, 0.7574803149606299524 ) ) ;
#30183=EDGE_CURVE ( 'NONE', #13348, #31518, #35680, .T. ) ;
#30215=FACE_BOUND ( 'NONE', #33927, .T. ) ;
#30247=EDGE_CURVE ( 'NONE', #29015, #44955, #18853, .T. ) ;
#30341=SURFACE_SIDE_STYLE ('',( #37243 ) ) ;
#30343=EDGE_LOOP ( 'NONE', ( #8853, #4832, #41777, #21234 ) ) ;
#30387=LINE ( 'NONE', #38008, #34651 ) ;
#30567=EDGE_LOOP ( 'NONE', ( #37857, #33337, #22420, #2637 ) ) ;
#30741=CARTESIAN_POINT ( 'NONE',  ( 0.8070866141732283561, -0.0009842519685049383633, 0.7574803149606299524 ) ) ;
#30762=SHAPE_REPRESENTATION ( 'Base Plate', ( #20860 ), #14766 ) ;
#30828=CARTESIAN_POINT ( 'NONE',  ( 0.8070866141732283561, 0.000000000000000000, -0.7574803149606299524 ) ) ;
#30851=CARTESIAN_POINT ( 'NONE',  ( 1.284448818897637956, 0.000000000000000000, 1.181102362204724310 ) ) ;
#30963=FACE_OUTER_BOUND ( 'NONE', #1546, .T. ) ;
#30965=CARTESIAN_POINT ( 'NONE',  ( -0.8070866141732283561, 0.000000000000000000, -0.8559055118110230342 ) ) ;
#31070=ADVANCED_FACE ( 'NONE', ( #1459 ), #41317, .F. ) ;
#31081=DIRECTION ( 'NONE',  ( 0.000000000000000000, 0.000000000000000000, 1.000000000000000000 ) ) ;
#31115=VERTEX_POINT ( 'NONE', #14846 ) ;
#31231=DIRECTION ( 'NONE',  ( -0.000000000000000000, 1.000000000000000000, -0.000000000000000000 ) ) ;
#31234=ADVANCED_FACE ( 'NONE', ( #7634 ), #21367, .F. ) ;
#31291=VERTEX_POINT ( 'NONE', #15315 ) ;
#31298=VECTOR ( 'NONE', #9759, 39.37007874015748143 ) ;
#31319=DIRECTION ( 'NONE',  ( 0.000000000000000000, 0.000000000000000000, 1.000000000000000000 ) ) ;
#31447=EDGE_LOOP ( 'NONE', ( #15854, #42712 ) ) ;
#31483=ORIENTED_EDGE ( 'NONE', *, *, #22725, .F. ) ;
#31518=VERTEX_POINT ( 'NONE', #36257 ) ;
#31699=LENGTH_MEASURE_WITH_UNIT ( LENGTH_MEASURE( 0.02539999999999999897 ), #46044 ) ;
#31711=DIMENSIONAL_EXPONENTS ( 1.000000000000000000, 0.000000000000000000, 0.000000000000000000, 0.000000000000000000, 0.000000000000000000, 0.000000000000000000, 0.000000000000000000 ) ;
#31720=EDGE_LOOP ( 'NONE', ( #33251, #37119 ) ) ;
#31759=ORIENTED_EDGE ( 'NONE', *, *, #22725, .T. ) ;
#31865=DIRECTION ( 'NONE',  ( 0.000000000000000000, 1.000000000000000000, 0.000000000000000000 ) ) ;
#31944=CIRCLE ( 'NONE', #5141, 0.09842519685039310962 ) ;
#32103=CONICAL_SURFACE ( 'NONE', #4481, 0.09842519685039310962, 0.7853981633972314524 ) ;
#32352=DIRECTION ( 'NONE',  ( 0.000000000000000000, -1.000000000000000000, -0.000000000000000000 ) ) ;
#32416=CARTESIAN_POINT ( 'NONE',  ( 0.8070866141732283561, 0.000000000000000000, -0.7574803149606299524 ) ) ;
#32536=CARTESIAN_POINT ( 'NONE',  ( -1.284448818897637956, -0.3937007874015748254, -1.181102362204724310 ) ) ;
#32544=ORIENTED_EDGE ( 'NONE', *, *, #3519, .T. ) ;
#32575=UNCERTAINTY_MEASURE_WITH_UNIT (LENGTH_MEASURE( 1.000000000000000082E-05 ), #46283, 'distance_accuracy_value', 'NONE') ;
#32629=VERTEX_POINT ( 'NONE', #34727 ) ;
#32652=DIRECTION ( 'NONE',  ( 0.000000000000000000, 0.000000000000000000, 1.000000000000000000 ) ) ;
#32786=CARTESIAN_POINT ( 'NONE',  ( -0.8070866141732283561, -0.3937007874015746034, 0.8559055118110230342 ) ) ;
#32806=VERTEX_POINT ( 'NONE', #32786 ) ;
#32821=DIRECTION ( 'NONE',  ( -0.000000000000000000, 1.000000000000000000, -0.000000000000000000 ) ) ;
#32847=CARTESIAN_POINT ( 'NONE',  ( -1.284448818897637956, 0.000000000000000000, 1.181102362204724310 ) ) ;
#32903=CARTESIAN_POINT ( 'NONE',  ( -0.8070866141732283561, 0.000000000000000000, -0.6580708661417323802 ) ) ;
#32947=EDGE_LOOP ( 'NONE', ( #17628, #46011 ) ) ;
#32993=ORIENTED_EDGE ( 'NONE', *, *, #34489, .T. ) ;
#33025=EDGE_LOOP ( 'NONE', ( #37447, #31759 ) ) ;
#33074=CIRCLE ( 'NONE', #12420, 0.09940944881889761386 ) ;
#33082=FACE_BOUND ( 'NONE', #31720, .T. ) ;
#33160=LINE ( 'NONE', #30965, #23928 ) ;
#33251=ORIENTED_EDGE ( 'NONE', *, *, #39533, .T. ) ;
#33260=CARTESIAN_POINT ( 'NONE',  ( 0.8070866141732283561, -0.0009842519685049383633, -0.7574803149606299524 ) ) ;
#33314=DIRECTION ( 'NONE',  ( -0.000000000000000000, 1.000000000000000000, -0.000000000000000000 ) ) ;
#33337=ORIENTED_EDGE ( 'NONE', *, *, #28155, .F. ) ;
#33472=DIRECTION ( 'NONE',  ( 1.000000000000000000, 0.000000000000000000, 0.000000000000000000 ) ) ;
#33483=DIRECTION ( 'NONE',  ( -1.000000000000000000, 0.000000000000000000, 0.000000000000000000 ) ) ;
#33550=DIRECTION ( 'NONE',  ( 0.000000000000000000, 0.000000000000000000, 1.000000000000000000 ) ) ;
#33689=FILL_AREA_STYLE ('',( #36785 ) ) ;
#33757=DIRECTION ( 'NONE',  ( -0.000000000000000000, 1.000000000000000000, -0.000000000000000000 ) ) ;
#33797=CARTESIAN_POINT ( 'NONE',  ( 0.000000000000000000, -0.3937007874015748254, 0.000000000000000000 ) ) ;
#33927=EDGE_LOOP ( 'NONE', ( #28613, #17092 ) ) ;
#33951=ORIENTED_EDGE ( 'NONE', *, *, #27705, .T. ) ;
#33998=DIRECTION ( 'NONE',  ( 8.659560562353054383E-17, 0.7071067811867007835, -0.7071067811863941399 ) ) ;
#34045=ORIENTED_EDGE ( 'NONE', *, *, #10681, .F. ) ;
#34069=VECTOR ( 'NONE', #34987, 39.37007874015748143 ) ;
#34141=ORIENTED_EDGE ( 'NONE', *, *, #29501, .T. ) ;
#34347=ORIENTED_EDGE ( 'NONE', *, *, #3519, .F. ) ;
#34361=CARTESIAN_POINT ( 'NONE',  ( 0.8070866141732283561, -0.0009842519685049383633, -0.8559055118110230342 ) ) ;
#34489=EDGE_CURVE ( 'NONE', #24250, #47218, #2571, .T. ) ;
#34587=CARTESIAN_POINT ( 'NONE',  ( 1.284448818897637956, 0.000000000000000000, -1.181102362204724310 ) ) ;
#34603=EDGE_LOOP ( 'NONE', ( #9407, #14629, #13497, #11049 ) ) ;
#34621=DIRECTION ( 'NONE',  ( 0.000000000000000000, -1.000000000000000000, -0.000000000000000000 ) ) ;
#34651=VECTOR ( 'NONE', #31081, 39.37007874015748143 ) ;
#34696=ORIENTED_EDGE ( 'NONE', *, *, #9710, .F. ) ;
#34703=ORIENTED_EDGE ( 'NONE', *, *, #18714, .F. ) ;
#34712=PRODUCT_DEFINITION_FORMATION_WITH_SPECIFIED_SOURCE ( 'ANY', '', #18798, .NOT_KNOWN. ) ;
#34727=CARTESIAN_POINT ( 'NONE',  ( 1.284448818897637956, 0.000000000000000000, 1.181102362204724310 ) ) ;
#34784=CONICAL_SURFACE ( 'NONE', #27165, 0.09842519685039310962, 0.7853981633972314524 ) ;
#34787=AXIS2_PLACEMENT_3D ( 'NONE', #28062, #45997, #46464 ) ;
#34883=FACE_OUTER_BOUND ( 'NONE', #16623, .T. ) ;
#34915=CARTESIAN_POINT ( 'NONE',  ( -0.8070866141732283561, -0.3937007874015746034, 0.7574803149606299524 ) ) ;
#34987=DIRECTION ( 'NONE',  ( -0.000000000000000000, 1.000000000000000000, -0.000000000000000000 ) ) ;
#35087=EDGE_LOOP ( 'NONE', ( #5205, #21834, #7494, #31483 ) ) ;
#35119=FACE_OUTER_BOUND ( 'NONE', #30343, .T. ) ;
#35221=CARTESIAN_POINT ( 'NONE',  ( 0.8070866141732283561, 0.000000000000000000, 0.6590551181102368705 ) ) ;
#35294=VECTOR ( 'NONE', #12507, 39.37007874015748854 ) ;
#35676=DIRECTION ( 'NONE',  ( 0.000000000000000000, 0.000000000000000000, 1.000000000000000000 ) ) ;
#35680=LINE ( 'NONE', #24885, #13782 ) ;
#35710=ADVANCED_FACE ( 'NONE', ( #27547 ), #12197, .F. ) ;
#35799=ORIENTED_EDGE ( 'NONE', *, *, #7901, .T. ) ;
#35862=LINE ( 'NONE', #17648, #11889 ) ;
#35885=CARTESIAN_POINT ( 'NONE',  ( 1.284448818897637956, -0.3937007874015748254, 1.181102362204724310 ) ) ;
#36042=ORIENTED_EDGE ( 'NONE', *, *, #27705, .F. ) ;
#36257=CARTESIAN_POINT ( 'NONE',  ( -0.8070866141732283561, -0.0009842519685049383633, 0.6590551181102368705 ) ) ;
#36286=VERTEX_POINT ( 'NONE', #23337 ) ;
#36292=VECTOR ( 'NONE', #11020, 39.37007874015748854 ) ;
#36412=ORIENTED_EDGE ( 'NONE', *, *, #27851, .T. ) ;
#36486=DIRECTION ( 'NONE',  ( -0.000000000000000000, 1.000000000000000000, -0.000000000000000000 ) ) ;
#36526=ORIENTED_EDGE ( 'NONE', *, *, #315, .F. ) ;
#36564=VECTOR ( 'NONE', #2813, 39.37007874015748143 ) ;
#36635=ORIENTED_EDGE ( 'NONE', *, *, #46027, .F. ) ;
#36669=CARTESIAN_POINT ( 'NONE',  ( -0.8070866141732283561, -0.0009842519685049383633, 0.7574803149606299524 ) ) ;
#36785=FILL_AREA_STYLE_COLOUR ( '', #38325 ) ;
#36792=CARTESIAN_POINT ( 'NONE',  ( 0.8070866141732283561, -0.3937007874015746034, 0.7574803149606299524 ) ) ;
#36823=PRODUCT_DEFINITION ( 'UNKNOWN', '', #34712, #2478 ) ;
#37017=( LENGTH_UNIT ( ) NAMED_UNIT ( * ) SI_UNIT ( $, .METRE. ) ) ;
#37084=PLANE ( 'NONE',  #15352 ) ;
#37108=DIRECTION ( 'NONE',  ( 0.000000000000000000, 0.000000000000000000, 1.000000000000000000 ) ) ;
#37119=ORIENTED_EDGE ( 'NONE', *, *, #10681, .T. ) ;
#37243=SURFACE_STYLE_FILL_AREA ( #33689 ) ;
#37257=VERTEX_POINT ( 'NONE', #47442 ) ;
#37335=DIRECTION ( 'NONE',  ( 0.000000000000000000, 1.000000000000000000, 0.000000000000000000 ) ) ;
#37447=ORIENTED_EDGE ( 'NONE', *, *, #315, .T. ) ;
#37453=DIRECTION ( 'NONE',  ( -1.000000000000000000, 0.000000000000000000, -0.000000000000000000 ) ) ;
#37497=ORIENTED_EDGE ( 'NONE', *, *, #10725, .F. ) ;
#37560=CARTESIAN_POINT ( 'NONE',  ( 0.000000000000000000, 0.000000000000000000, 0.000000000000000000 ) ) ;
#37580=DIRECTION ( 'NONE',  ( -0.000000000000000000, 1.000000000000000000, -0.000000000000000000 ) ) ;
#37686=DIRECTION ( 'NONE',  ( 0.000000000000000000, 0.000000000000000000, 1.000000000000000000 ) ) ;
#37857=ORIENTED_EDGE ( 'NONE', *, *, #8571, .F. ) ;
#37859=AXIS2_PLACEMENT_3D ( 'NONE', #38200, #34621, #1771 ) ;
#37868=CARTESIAN_POINT ( 'NONE',  ( 0.8070866141732283561, -0.0009842519685049383633, -0.7574803149606299524 ) ) ;
#37874=LINE ( 'NONE', #19649, #39387 ) ;
#37987=CARTESIAN_POINT ( 'NONE',  ( -0.8070866141732283561, -0.0009842519685049383633, -0.7574803149606299524 ) ) ;
#38008=CARTESIAN_POINT ( 'NONE',  ( -1.284448818897637956, 0.000000000000000000, -1.181102362204724310 ) ) ;
#38055=DIRECTION ( 'NONE',  ( 0.000000000000000000, 0.7071067811867007835, 0.7071067811863941399 ) ) ;
#38200=CARTESIAN_POINT ( 'NONE',  ( -0.8070866141732283561, 0.000000000000000000, 0.7574803149606299524 ) ) ;
#38218=VECTOR ( 'NONE', #43176, 39.37007874015748143 ) ;
#38243=DIRECTION ( 'NONE',  ( -0.000000000000000000, 1.000000000000000000, -0.000000000000000000 ) ) ;
#38280=ORIENTED_EDGE ( 'NONE', *, *, #7797, .T. ) ;
#38282=CIRCLE ( 'NONE', #17621, 0.09842519685039310962 ) ;
#38325=COLOUR_RGB ( '', 0.09019608, 0.27058824, 0.51372549) ;
#38338=EDGE_LOOP ( 'NONE', ( #27023, #36412, #44943, #32544 ) ) ;
#38401=DIRECTION ( 'NONE',  ( 0.000000000000000000, 0.000000000000000000, 1.000000000000000000 ) ) ;
#38454=FACE_OUTER_BOUND ( 'NONE', #43759, .T. ) ;
#38461=ORIENTED_EDGE ( 'NONE', *, *, #43540, .T. ) ;
#38562=EDGE_LOOP ( 'NONE', ( #15897, #45318, #37497, #43279 ) ) ;
#38563=ORIENTED_EDGE ( 'NONE', *, *, #28155, .T. ) ;
#38640=CARTESIAN_POINT ( 'NONE',  ( -0.8070866141732283561, -0.0009842519685049383633, -0.7574803149606299524 ) ) ;
#38775=CARTESIAN_POINT ( 'NONE',  ( 0.8070866141732283561, -0.3937007874015746034, 0.6590551181102368705 ) ) ;
#38781=DIRECTION ( 'NONE',  ( -0.000000000000000000, 1.000000000000000000, -0.000000000000000000 ) ) ;
#39013=DIRECTION ( 'NONE',  ( 0.000000000000000000, 1.000000000000000000, 0.000000000000000000 ) ) ;
#39233=CARTESIAN_POINT ( 'NONE',  ( 0.8070866141732283561, 0.000000000000000000, -0.6590551181102368705 ) ) ;
#39325=DIRECTION ( 'NONE',  ( 0.000000000000000000, -1.000000000000000000, -0.000000000000000000 ) ) ;
#39329=DIRECTION ( 'NONE',  ( -0.000000000000000000, 1.000000000000000000, -0.000000000000000000 ) ) ;
#39387=VECTOR ( 'NONE', #44554, 39.37007874015748143 ) ;
#39406=DIRECTION ( 'NONE',  ( -0.000000000000000000, 1.000000000000000000, -0.000000000000000000 ) ) ;
#39409=CARTESIAN_POINT ( 'NONE',  ( -0.8070866141732283561, -0.0009842519685049383633, -0.6590551181102368705 ) ) ;
#39477=CARTESIAN_POINT ( 'NONE',  ( 1.284448818897637956, -0.3937007874015748254, -1.181102362204724310 ) ) ;
#39533=EDGE_CURVE ( 'NONE', #24250, #20094, #21118, .T. ) ;
#39584=VERTEX_POINT ( 'NONE', #32903 ) ;
#39585=LINE ( 'NONE', #20200, #38218 ) ;
#39801=AXIS2_PLACEMENT_3D ( 'NONE', #30115, #23117, #29647 ) ;
#39837=VERTEX_POINT ( 'NONE', #38775 ) ;
#39910=ORIENTED_EDGE ( 'NONE', *, *, #41961, .F. ) ;
#40144=LINE ( 'NONE', #42777, #22724 ) ;
#40345=LINE ( 'NONE', #11385, #21215 ) ;
#40391=DIRECTION ( 'NONE',  ( 0.000000000000000000, 0.000000000000000000, 1.000000000000000000 ) ) ;
#40433=CYLINDRICAL_SURFACE ( 'NONE', #7289, 0.09842519685039310962 ) ;
#40445=CARTESIAN_POINT ( 'NONE',  ( -0.8070866141732283561, -0.0009842519685049383633, -0.7574803149606299524 ) ) ;
#40501=EDGE_CURVE ( 'NONE', #3834, #32629, #30103, .T. ) ;
#40738=LINE ( 'NONE', #7933, #35294 ) ;
#40749=CARTESIAN_POINT ( 'NONE',  ( 0.8070866141732283561, -0.3937007874015746034, 0.8559055118110230342 ) ) ;
#40892=FACE_BOUND ( 'NONE', #17551, .T. ) ;
#40941=DIRECTION ( 'NONE',  ( 0.000000000000000000, -1.000000000000000000, -0.000000000000000000 ) ) ;
#40951=AXIS2_PLACEMENT_3D ( 'NONE', #7396, #32352, #46930 ) ;
#40952=CARTESIAN_POINT ( 'NONE',  ( -0.8070866141732283561, 0.000000000000000000, 0.8568897637795275246 ) ) ;
#40958=DIRECTION ( 'NONE',  ( 8.659560562353054383E-17, 0.7071067811867007835, -0.7071067811863941399 ) ) ;
#40992=DIRECTION ( 'NONE',  ( 0.000000000000000000, -1.000000000000000000, -0.000000000000000000 ) ) ;
#41041=CARTESIAN_POINT ( 'NONE',  ( 1.284448818897637956, -0.3937007874015748254, 1.181102362204724310 ) ) ;
#41077=ORIENTED_EDGE ( 'NONE', *, *, #16885, .T. ) ;
#41317=CONICAL_SURFACE ( 'NONE', #6143, 0.09842519685039310962, 0.7853981633972314524 ) ;
#41362=( GEOMETRIC_REPRESENTATION_CONTEXT ( 3 ) GLOBAL_UNCERTAINTY_ASSIGNED_CONTEXT ( ( #8130 ) ) GLOBAL_UNIT_ASSIGNED_CONTEXT ( ( #44890, #29417, #43962 ) ) REPRESENTATION_CONTEXT ( 'NONE', 'WORKASPACE' ) ) ;
#41383=CARTESIAN_POINT ( 'NONE',  ( -0.8070866141732283561, -0.0009842519685049383633, 0.7574803149606299524 ) ) ;
#41567=ADVANCED_FACE ( 'NONE', ( #8677 ), #1080, .F. ) ;
#41619=ORIENTED_EDGE ( 'NONE', *, *, #30183, .F. ) ;
#41653=LINE ( 'NONE', #35221, #34069 ) ;
#41694=DIRECTION ( 'NONE',  ( 0.000000000000000000, 0.000000000000000000, -1.000000000000000000 ) ) ;
#41777=ORIENTED_EDGE ( 'NONE', *, *, #46677, .F. ) ;
#41893=AXIS2_PLACEMENT_3D ( 'NONE', #10585, #29538, #22280 ) ;
#41961=EDGE_CURVE ( 'NONE', #39584, #11722, #4195, .T. ) ;
#41983=DIRECTION ( 'NONE',  ( 0.000000000000000000, -1.000000000000000000, -0.000000000000000000 ) ) ;
#42099=CARTESIAN_POINT ( 'NONE',  ( 0.8070866141732283561, 0.000000000000000000, 0.7574803149606299524 ) ) ;
#42134=DIRECTION ( 'NONE',  ( 0.000000000000000000, 0.000000000000000000, 1.000000000000000000 ) ) ;
#42272=DIRECTION ( 'NONE',  ( -0.000000000000000000, 1.000000000000000000, -0.000000000000000000 ) ) ;
#42275=ORIENTED_EDGE ( 'NONE', *, *, #43745, .F. ) ;
#42334=ORIENTED_EDGE ( 'NONE', *, *, #10243, .F. ) ;
#42468=AXIS2_PLACEMENT_3D ( 'NONE', #26803, #20297, #16485 ) ;
#42647=ADVANCED_FACE ( 'NONE', ( #2206 ), #13257, .F. ) ;
#42665=( NAMED_UNIT ( * ) PLANE_ANGLE_UNIT ( ) SI_UNIT ( $, .RADIAN. ) ) ;
#42712=ORIENTED_EDGE ( 'NONE', *, *, #4811, .T. ) ;
#42716=ADVANCED_FACE ( 'NONE', ( #24270 ), #400, .F. ) ;
#42777=CARTESIAN_POINT ( 'NONE',  ( -0.8070866141732283561, -0.0009842519685049383633, -0.8559055118110230342 ) ) ;
#42997=DIRECTION ( 'NONE',  ( 0.000000000000000000, 0.7071067811867007835, 0.7071067811863941399 ) ) ;
#43115=ORIENTED_EDGE ( 'NONE', *, *, #28716, .T. ) ;
#43133=CARTESIAN_POINT ( 'NONE',  ( -0.8070866141732283561, 0.000000000000000000, -0.8568897637795275246 ) ) ;
#43176=DIRECTION ( 'NONE',  ( 0.000000000000000000, 1.000000000000000000, 0.000000000000000000 ) ) ;
#43217=AXIS2_PLACEMENT_3D ( 'NONE', #30000, #40941, #8136 ) ;
#43266=AXIS2_PLACEMENT_3D ( 'NONE', #37560, #12174, #26798 ) ;
#43279=ORIENTED_EDGE ( 'NONE', *, *, #13405, .F. ) ;
#43394=CARTESIAN_POINT ( 'NONE',  ( -0.8070866141732283561, -0.3937007874015746034, -0.7574803149606299524 ) ) ;
#43403=CIRCLE ( 'NONE', #22008, 0.09842519685039310962 ) ;
#43494=ORIENTED_EDGE ( 'NONE', *, *, #13405, .T. ) ;
#43540=EDGE_CURVE ( 'NONE', #31291, #2480, #6628, .T. ) ;
#43629=SHAPE_REPRESENTATION_RELATIONSHIP ( 'NONE' , 'NONE' ,  #30762, #27401 ) ;
#43646=AXIS2_PLACEMENT_3D ( 'NONE', #30828, #42272, #23606 ) ;
#43745=EDGE_CURVE ( 'NONE', #27408, #10456, #11838, .T. ) ;
#43759=EDGE_LOOP ( 'NONE', ( #36042, #13698, #32993, #38563 ) ) ;
#43819=CARTESIAN_POINT ( 'NONE',  ( -0.8070866141732283561, -0.0009842519685049383633, 0.6590551181102368705 ) ) ;
#43962=( NAMED_UNIT ( * ) SI_UNIT ( $, .STERADIAN. ) SOLID_ANGLE_UNIT ( ) ) ;
#43993=EDGE_LOOP ( 'NONE', ( #41619, #3451, #13360, #26679 ) ) ;
#44065=LINE ( 'NONE', #32847, #27448 ) ;
#44100=CARTESIAN_POINT ( 'NONE',  ( 0.8070866141732283561, -0.0009842519685049383633, -0.6590551181102368705 ) ) ;
#44513=LINE ( 'NONE', #43819, #36292 ) ;
#44518=VECTOR ( 'NONE', #38055, 39.37007874015748854 ) ;
#44554=DIRECTION ( 'NONE',  ( 0.000000000000000000, 1.000000000000000000, 0.000000000000000000 ) ) ;
#44670=EDGE_CURVE ( 'NONE', #32806, #36286, #35862, .T. ) ;
#44760=FACE_BOUND ( 'NONE', #32947, .T. ) ;
#44889=ORIENTED_EDGE ( 'NONE', *, *, #9710, .T. ) ;
#44890=( CONVERSION_BASED_UNIT ( 'INCH', #3941 ) LENGTH_UNIT ( ) NAMED_UNIT ( #31711 ) ) ;
#44943=ORIENTED_EDGE ( 'NONE', *, *, #43745, .T. ) ;
#44955=VERTEX_POINT ( 'NONE', #889 ) ;
#44963=FACE_BOUND ( 'NONE', #29443, .T. ) ;
#44990=FACE_OUTER_BOUND ( 'NONE', #4170, .T. ) ;
#45175=LINE ( 'NONE', #30851, #28243 ) ;
#45206=VECTOR ( 'NONE', #42997, 39.37007874015748854 ) ;
#45279=AXIS2_PLACEMENT_3D ( 'NONE', #14005, #21672, #21907 ) ;
#45310=AXIS2_PLACEMENT_3D ( 'NONE', #26425, #40992, #10869 ) ;
#45318=ORIENTED_EDGE ( 'NONE', *, *, #7797, .F. ) ;
#45323=ADVANCED_FACE ( 'NONE', ( #17891 ), #15029, .T. ) ;
#45341=CARTESIAN_POINT ( 'NONE',  ( 0.8070866141732283561, 0.000000000000000000, -0.7574803149606299524 ) ) ;
#45486=EDGE_LOOP ( 'NONE', ( #12373, #36635, #38461, #26976 ) ) ;
#45630=DIRECTION ( 'NONE',  ( 0.000000000000000000, 0.000000000000000000, 1.000000000000000000 ) ) ;
#45749=DIMENSIONAL_EXPONENTS ( 1.000000000000000000, 0.000000000000000000, 0.000000000000000000, 0.000000000000000000, 0.000000000000000000, 0.000000000000000000, 0.000000000000000000 ) ;
#45753=ADVANCED_FACE ( 'NONE', ( #35119 ), #46792, .F. ) ;
#45866=ORIENTED_EDGE ( 'NONE', *, *, #30247, .F. ) ;
#45997=DIRECTION ( 'NONE',  ( 0.000000000000000000, -1.000000000000000000, -0.000000000000000000 ) ) ;
#46011=ORIENTED_EDGE ( 'NONE', *, *, #4150, .T. ) ;
#46027=EDGE_CURVE ( 'NONE', #31291, #1170, #28493, .T. ) ;
#46044=( LENGTH_UNIT ( ) NAMED_UNIT ( * ) SI_UNIT ( $, .METRE. ) ) ;
#46049=DIRECTION ( 'NONE',  ( 0.000000000000000000, 1.000000000000000000, 0.000000000000000000 ) ) ;
#46200=LINE ( 'NONE', #39477, #36564 ) ;
#46217=CIRCLE ( 'NONE', #34787, 0.09940944881889761386 ) ;
#46283=( CONVERSION_BASED_UNIT ( 'INCH', #31699 ) LENGTH_UNIT ( ) NAMED_UNIT ( #45749 ) ) ;
#46438=ORIENTED_EDGE ( 'NONE', *, *, #5744, .F. ) ;
#46464=DIRECTION ( 'NONE',  ( 0.000000000000000000, 0.000000000000000000, 1.000000000000000000 ) ) ;
#46677=EDGE_CURVE ( 'NONE', #37257, #25961, #33074, .T. ) ;
#46692=ORIENTED_EDGE ( 'NONE', *, *, #10359, .T. ) ;
#46792=CONICAL_SURFACE ( 'NONE', #14653, 0.09842519685039310962, 0.7853981633972314524 ) ;
#46842=EDGE_CURVE ( 'NONE', #36286, #5716, #22967, .T. ) ;
#46869=LINE ( 'NONE', #14054, #31298 ) ;
#46930=DIRECTION ( 'NONE',  ( 0.000000000000000000, 0.000000000000000000, 1.000000000000000000 ) ) ;
#47218=VERTEX_POINT ( 'NONE', #16138 ) ;
#47325=VECTOR ( 'NONE', #4078, 39.37007874015748854 ) ;
#47409=CARTESIAN_POINT ( 'NONE',  ( 0.8070866141732283561, -0.3937007874015746034, -0.6590551181102368705 ) ) ;
#47442=CARTESIAN_POINT ( 'NONE',  ( 0.8070866141732283561, 0.000000000000000000, -0.6580708661417323802 ) ) ;
ENDSEC;
END-ISO-10303-21;
